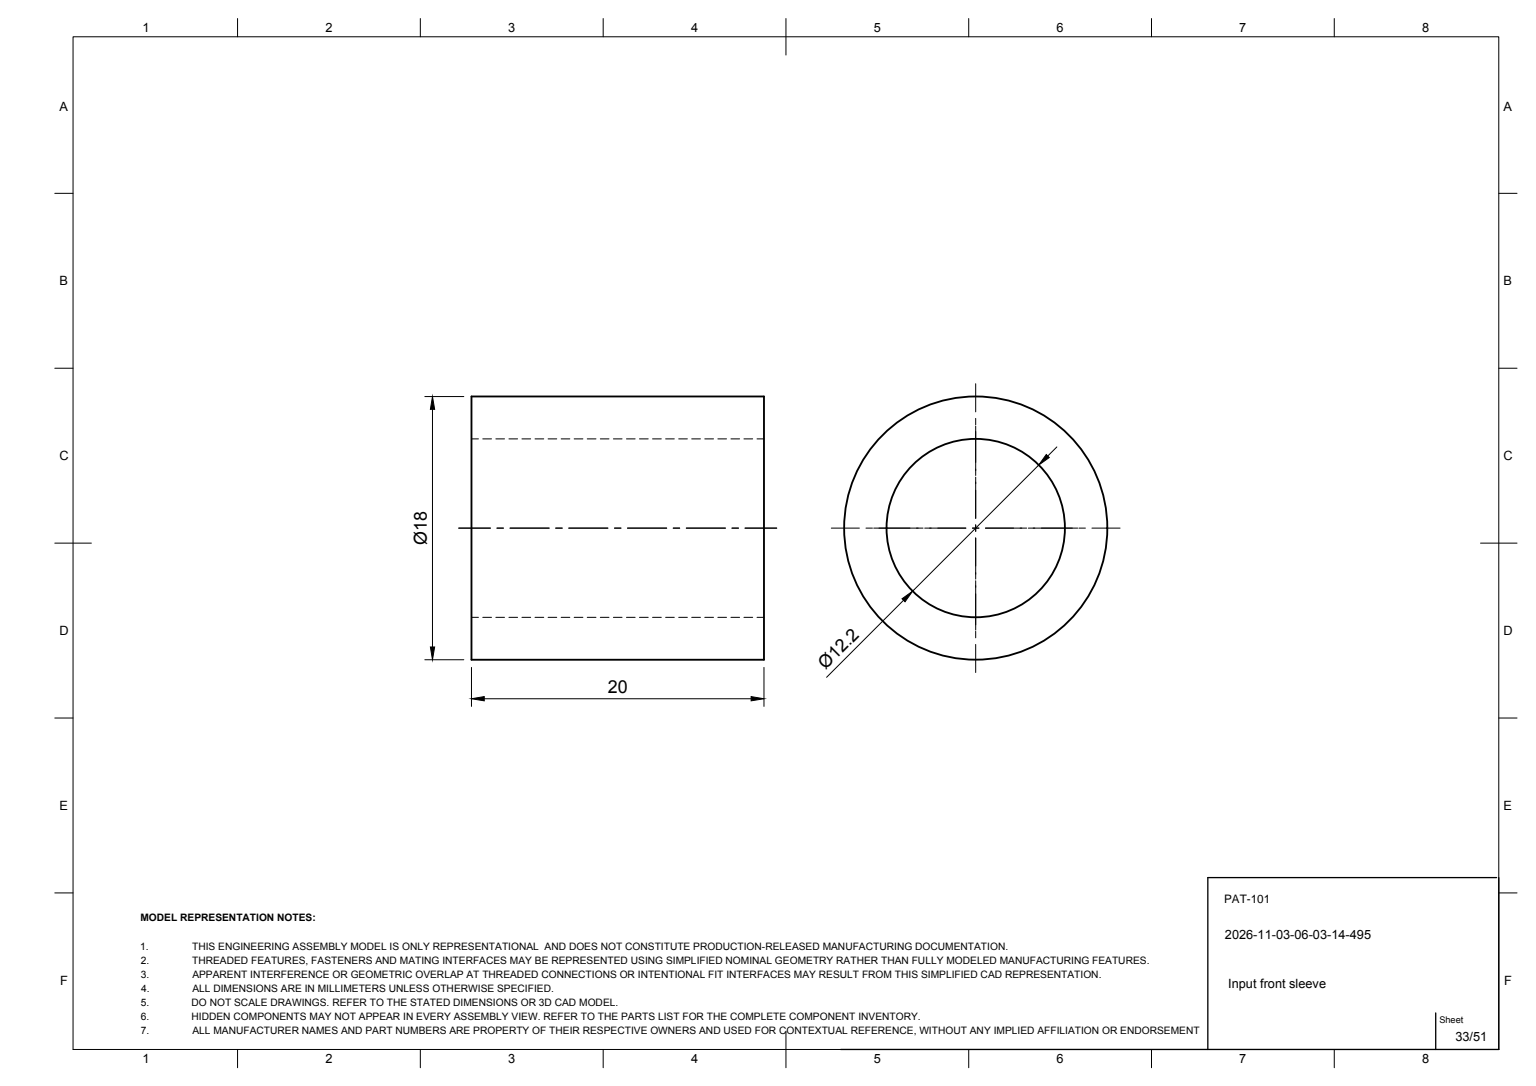
ISO-10303-21;
HEADER;
/* Generated by software containing ST-Developer
 * from STEP Tools, Inc. (www.steptools.com) 
 */

FILE_DESCRIPTION(
/* description */ ('Spur gear reduction stage 2-1 on bearing plates'),
/* implementation_level */ '2;1');

FILE_NAME(
/* name */ 'Input front sleeve.step',
/* time_stamp */ '2026-10-28T03:22:07-07:00',
/* author */ (''),
/* organization */ (''),
/* preprocessor_version */ 'ST-DEVELOPER v20.2',
/* originating_system */ 'Autodesk Translation Framework v15.17.0.0',
/* authorisation */ '');

FILE_SCHEMA (('AUTOMOTIVE_DESIGN { 1 0 10303 214 3 1 1 }'));
ENDSEC;

DATA;
#10=MECHANICAL_DESIGN_GEOMETRIC_PRESENTATION_REPRESENTATION('',(#987),#53909);
#886=SHAPE_REPRESENTATION_RELATIONSHIP('SRR','None',#54116,#929);
#929=ADVANCED_BREP_SHAPE_REPRESENTATION('',(#1042),#53890);
#987=STYLED_ITEM('',(#54383),#1042);
#1042=MANIFOLD_SOLID_BREP('Body1',#11314);
#1198=FACE_BOUND('',#2580,.T.);
#1199=FACE_BOUND('',#2582,.T.);
#1365=PLANE('',#12501);
#1366=PLANE('',#12502);
#1791=FACE_OUTER_BOUND('',#2577,.T.);
#1792=FACE_OUTER_BOUND('',#2578,.T.);
#1793=FACE_OUTER_BOUND('',#2579,.T.);
#1794=FACE_OUTER_BOUND('',#2581,.T.);
#2577=EDGE_LOOP('',(#8512,#8513,#8514,#8515));
#2578=EDGE_LOOP('',(#8516,#8517,#8518,#8519));
#2579=EDGE_LOOP('',(#8520));
#2580=EDGE_LOOP('',(#8521));
#2581=EDGE_LOOP('',(#8522));
#2582=EDGE_LOOP('',(#8523));
#3204=LINE('',#17959,#3845);
#3205=LINE('',#17965,#3846);
#3845=VECTOR('',#14591,0.61);
#3846=VECTOR('',#14598,0.9);
#4580=CIRCLE('',#12496,0.61);
#4581=CIRCLE('',#12497,0.61);
#4582=CIRCLE('',#12499,0.9);
#4583=CIRCLE('',#12500,0.9);
#5184=VERTEX_POINT('',#17956);
#5185=VERTEX_POINT('',#17958);
#5186=VERTEX_POINT('',#17962);
#5187=VERTEX_POINT('',#17964);
#6398=EDGE_CURVE('',#5184,#5184,#4580,.T.);
#6399=EDGE_CURVE('',#5184,#5185,#3204,.T.);
#6400=EDGE_CURVE('',#5185,#5185,#4581,.T.);
#6401=EDGE_CURVE('',#5186,#5186,#4582,.T.);
#6402=EDGE_CURVE('',#5186,#5187,#3205,.T.);
#6403=EDGE_CURVE('',#5187,#5187,#4583,.T.);
#8512=ORIENTED_EDGE('',*,*,#6398,.F.);
#8513=ORIENTED_EDGE('',*,*,#6399,.T.);
#8514=ORIENTED_EDGE('',*,*,#6400,.T.);
#8515=ORIENTED_EDGE('',*,*,#6399,.F.);
#8516=ORIENTED_EDGE('',*,*,#6401,.F.);
#8517=ORIENTED_EDGE('',*,*,#6402,.T.);
#8518=ORIENTED_EDGE('',*,*,#6403,.T.);
#8519=ORIENTED_EDGE('',*,*,#6402,.F.);
#8520=ORIENTED_EDGE('',*,*,#6401,.T.);
#8521=ORIENTED_EDGE('',*,*,#6398,.T.);
#8522=ORIENTED_EDGE('',*,*,#6403,.F.);
#8523=ORIENTED_EDGE('',*,*,#6400,.F.);
#10527=CYLINDRICAL_SURFACE('',#12495,0.61);
#10528=CYLINDRICAL_SURFACE('',#12498,0.9);
#10911=ADVANCED_FACE('',(#1791),#10527,.F.);
#10912=ADVANCED_FACE('',(#1792),#10528,.T.);
#10913=ADVANCED_FACE('',(#1793,#1198),#1365,.T.);
#10914=ADVANCED_FACE('',(#1794,#1199),#1366,.F.);
#11314=CLOSED_SHELL('',(#10911,#10912,#10913,#10914));
#12494=AXIS2_PLACEMENT_3D('',#17954,#14585,#14586);
#12495=AXIS2_PLACEMENT_3D('',#17955,#14587,#14588);
#12496=AXIS2_PLACEMENT_3D('',#17957,#14589,#14590);
#12497=AXIS2_PLACEMENT_3D('',#17960,#14592,#14593);
#12498=AXIS2_PLACEMENT_3D('',#17961,#14594,#14595);
#12499=AXIS2_PLACEMENT_3D('',#17963,#14596,#14597);
#12500=AXIS2_PLACEMENT_3D('',#17966,#14599,#14600);
#12501=AXIS2_PLACEMENT_3D('',#17967,#14601,#14602);
#12502=AXIS2_PLACEMENT_3D('',#17968,#14603,#14604);
#14585=DIRECTION('axis',(0.,0.,1.));
#14586=DIRECTION('refdir',(1.,0.,0.));
#14587=DIRECTION('center_axis',(0.,1.,0.));
#14588=DIRECTION('ref_axis',(1.,0.,0.));
#14589=DIRECTION('center_axis',(0.,-1.,0.));
#14590=DIRECTION('ref_axis',(1.,0.,0.));
#14591=DIRECTION('',(0.,-1.,0.));
#14592=DIRECTION('center_axis',(0.,-1.,0.));
#14593=DIRECTION('ref_axis',(1.,0.,0.));
#14594=DIRECTION('center_axis',(0.,1.,0.));
#14595=DIRECTION('ref_axis',(1.,0.,0.));
#14596=DIRECTION('center_axis',(0.,1.,0.));
#14597=DIRECTION('ref_axis',(1.,0.,0.));
#14598=DIRECTION('',(0.,-1.,0.));
#14599=DIRECTION('center_axis',(0.,1.,0.));
#14600=DIRECTION('ref_axis',(1.,0.,0.));
#14601=DIRECTION('center_axis',(0.,1.,0.));
#14602=DIRECTION('ref_axis',(1.,0.,0.));
#14603=DIRECTION('center_axis',(0.,1.,0.));
#14604=DIRECTION('ref_axis',(1.,0.,0.));
#17954=CARTESIAN_POINT('',(0.,0.,0.));
#17955=CARTESIAN_POINT('Origin',(0.,-3.,0.));
#17956=CARTESIAN_POINT('',(-0.61,-1.,7.47034547479885E-17));
#17957=CARTESIAN_POINT('Origin',(0.,-1.,0.));
#17958=CARTESIAN_POINT('',(-0.61,-3.,7.47034547479885E-17));
#17959=CARTESIAN_POINT('',(-0.61,-3.,7.47034547479885E-17));
#17960=CARTESIAN_POINT('Origin',(0.,-3.,0.));
#17961=CARTESIAN_POINT('Origin',(0.,-3.,0.));
#17962=CARTESIAN_POINT('',(-0.9,-1.,1.10218211923262E-16));
#17963=CARTESIAN_POINT('Origin',(0.,-1.,0.));
#17964=CARTESIAN_POINT('',(-0.9,-3.,1.10218211923262E-16));
#17965=CARTESIAN_POINT('',(-0.9,-3.,1.10218211923262E-16));
#17966=CARTESIAN_POINT('Origin',(0.,-3.,0.));
#17967=CARTESIAN_POINT('Origin',(0.,-1.,0.));
#17968=CARTESIAN_POINT('Origin',(0.,-3.,0.));
#53840=UNCERTAINTY_MEASURE_WITH_UNIT(LENGTH_MEASURE(0.001),#53910,
'DISTANCE_ACCURACY_VALUE',
'Maximum model space distance between geometric entities at asserted c
onnectivities');
#53859=UNCERTAINTY_MEASURE_WITH_UNIT(LENGTH_MEASURE(0.001),#53910,
'DISTANCE_ACCURACY_VALUE',
'Maximum model space distance between geometric entities at asserted c
onnectivities');
#53890=(
GEOMETRIC_REPRESENTATION_CONTEXT(3)
GLOBAL_UNCERTAINTY_ASSIGNED_CONTEXT((#53840))
GLOBAL_UNIT_ASSIGNED_CONTEXT((#53910,#53912,#53913))
REPRESENTATION_CONTEXT('','3D')
);
#53909=(
GEOMETRIC_REPRESENTATION_CONTEXT(3)
GLOBAL_UNCERTAINTY_ASSIGNED_CONTEXT((#53859))
GLOBAL_UNIT_ASSIGNED_CONTEXT((#53910,#53912,#53913))
REPRESENTATION_CONTEXT('','3D')
);
#53910=(
LENGTH_UNIT()
NAMED_UNIT(*)
SI_UNIT(.CENTI.,.METRE.)
);
#53912=(
NAMED_UNIT(*)
PLANE_ANGLE_UNIT()
SI_UNIT($,.RADIAN.)
);
#53913=(
NAMED_UNIT(*)
SI_UNIT($,.STERADIAN.)
SOLID_ANGLE_UNIT()
);
#53944=SHAPE_DEFINITION_REPRESENTATION(#54042,#54116);
#54042=PRODUCT_DEFINITION_SHAPE('',$,#54166);
#54116=SHAPE_REPRESENTATION('',(#12494),#53890);
#54135=PRODUCT_DEFINITION_CONTEXT('part definition',#54284,'design');
#54166=PRODUCT_DEFINITION('Input front sleeve','Input front sleeve',#54215,
#54135);
#54215=PRODUCT_DEFINITION_FORMATION('',$,#54316);
#54284=APPLICATION_CONTEXT(
'Core Data for Automotive Mechanical Design Process');
#54285=PRODUCT_CONTEXT('part definition',#54284,'mechanical');
#54316=PRODUCT('Input front sleeve','Input front sleeve',
'Input front sleeve',(#54285));
#54377=COLOUR_RGB('Light Blue',0.38,0.62,0.78);
#54378=FILL_AREA_STYLE_COLOUR('',#54377);
#54379=FILL_AREA_STYLE('',(#54378));
#54380=SURFACE_STYLE_FILL_AREA(#54379);
#54381=SURFACE_SIDE_STYLE('',(#54380));
#54382=SURFACE_STYLE_USAGE(.BOTH.,#54381);
#54383=PRESENTATION_STYLE_ASSIGNMENT((#54382));
ENDSEC;
END-ISO-10303-21;
